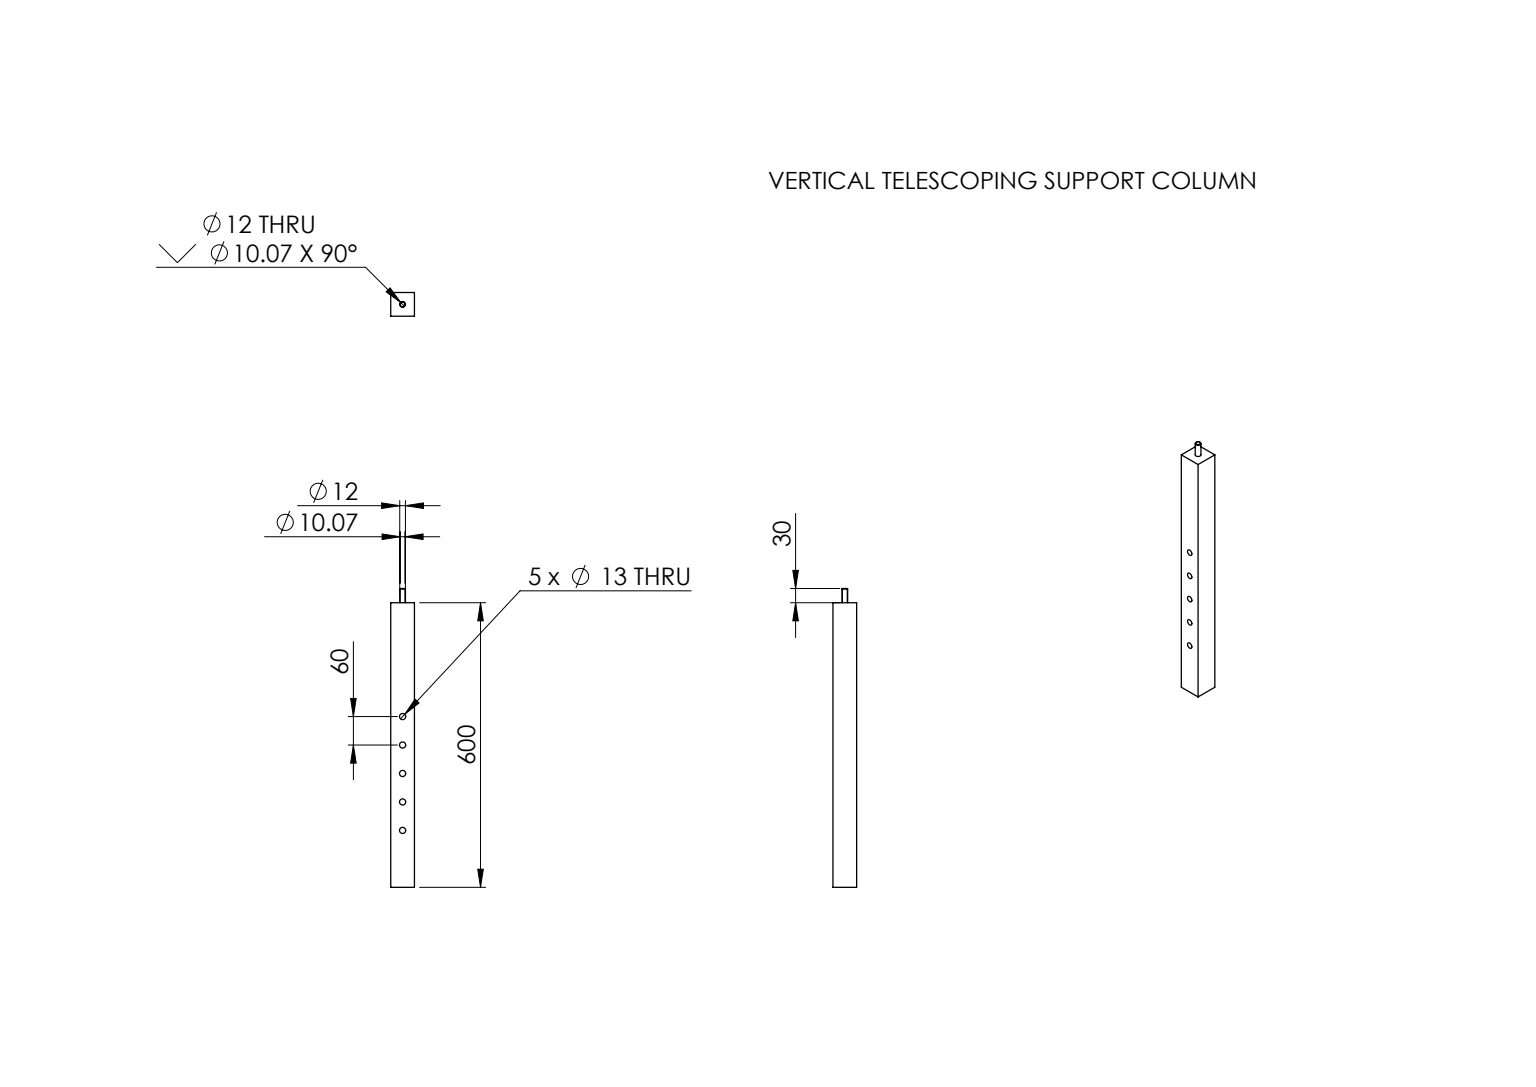
ISO-10303-21;
HEADER;
FILE_DESCRIPTION (('STEP AP214'),
    '1' );
FILE_NAME ('Vertical Telescoping Support Column.step',
    '2026-10-22T16:49:52',
    ( '' ),
    ( '' ),
    'SwSTEP 2.0',
    'SolidWorks 2026',
    '' );
FILE_SCHEMA (( 'AUTOMOTIVE_DESIGN' ));
ENDSEC;

DATA;
#19=APPLICATION_CONTEXT ( 'automotive_design' ) ;
#32=DIRECTION ( 'NONE',  ( 1.000000000000000000, -0.000000000000000000, 6.938893903907228378E-17 ) ) ;
#61=CARTESIAN_POINT ( 'NONE',  ( -24.99999999999999645, 810.0000000000000000, -25.00000000000000000 ) ) ;
#66=EDGE_LOOP ( 'NONE', ( #727, #5386, #2171, #4175 ) ) ;
#70=VECTOR ( 'NONE', #4320, 1000.000000000000000 ) ;
#84=DIRECTION ( 'NONE',  ( 2.081668171172168513E-16, 0.000000000000000000, -1.000000000000000000 ) ) ;
#89=DIRECTION ( 'NONE',  ( 1.000000000000000000, 0.000000000000000000, 0.000000000000000000 ) ) ;
#95=UNCERTAINTY_MEASURE_WITH_UNIT (LENGTH_MEASURE( 1.000000000000000082E-05 ), #3819, 'distance_accuracy_value', 'NONE');
#97=CARTESIAN_POINT ( 'NONE',  ( 0.000000000000000000, 810.0000000000000000, 0.000000000000000000 ) ) ;
#119=ADVANCED_BREP_SHAPE_REPRESENTATION ( '', ( #1812, #4154 ), #5370 ) ;
#127=DIRECTION ( 'NONE',  ( -0.000000000000000000, -0.000000000000000000, 1.000000000000000000 ) ) ;
#128=VECTOR ( 'NONE', #1979, 1000.000000000000000 ) ;
#129=CIRCLE ( 'NONE', #3889, 6.000000000000000000 ) ;
#151=ORIENTED_EDGE ( 'NONE', *, *, #3972, .F. ) ;
#161=ORIENTED_EDGE ( 'NONE', *, *, #5198, .T. ) ;
#164=DIRECTION ( 'NONE',  ( -0.000000000000000000, -0.000000000000000000, 1.000000000000000000 ) ) ;
#181=CARTESIAN_POINT ( 'NONE',  ( 0.000000000000000000, 450.0000000000000000, 25.00000000000000000 ) ) ;
#186=LINE ( 'NONE', #5103, #588 ) ;
#194=EDGE_CURVE ( 'NONE', #2394, #3572, #803, .T. ) ;
#200=ORIENTED_EDGE ( 'NONE', *, *, #4627, .T. ) ;
#204=CARTESIAN_POINT ( 'NONE',  ( 0.000000000000000000, 450.0000000000000000, -25.00000000000000000 ) ) ;
#210=CARTESIAN_POINT ( 'NONE',  ( 5.035999999999999588, 840.0000000000001137, 0.000000000000000000 ) ) ;
#217=CIRCLE ( 'NONE', #2845, 6.499999999999988454 ) ;
#223=ADVANCED_FACE ( 'NONE', ( #720 ), #3527, .F. ) ;
#226=CIRCLE ( 'NONE', #1785, 6.499999999999988454 ) ;
#237=ADVANCED_FACE ( 'NONE', ( #3202, #2295 ), #602, .T. ) ;
#253=DIRECTION ( 'NONE',  ( 1.000000000000000000, 0.000000000000000000, 0.000000000000000000 ) ) ;
#269=DIRECTION ( 'NONE',  ( 0.000000000000000000, 0.000000000000000000, -1.000000000000000000 ) ) ;
#271=CARTESIAN_POINT ( 'NONE',  ( 6.499999999999988454, 450.0000000000000000, -25.00000000000000000 ) ) ;
#325=VECTOR ( 'NONE', #1251, 1000.000000000000000 ) ;
#355=CARTESIAN_POINT ( 'NONE',  ( 0.000000000000000000, 810.0000000000000000, 0.000000000000000000 ) ) ;
#356=DIRECTION ( 'NONE',  ( 0.000000000000000000, -0.000000000000000000, 1.000000000000000000 ) ) ;
#357=DIRECTION ( 'NONE',  ( 1.000000000000000000, 0.000000000000000000, 0.000000000000000000 ) ) ;
#364=DIRECTION ( 'NONE',  ( 0.000000000000000000, 0.000000000000000000, -1.000000000000000000 ) ) ;
#393=CARTESIAN_POINT ( 'NONE',  ( -6.499999999999988454, 330.0000000000000000, 25.00000000000000000 ) ) ;
#396=ORIENTED_EDGE ( 'NONE', *, *, #1896, .F. ) ;
#398=EDGE_LOOP ( 'NONE', ( #3947, #1847, #2985, #1194 ) ) ;
#408=ADVANCED_FACE ( 'NONE', ( #4526 ), #855, .T. ) ;
#423=AXIS2_PLACEMENT_3D ( 'NONE', #2818, #3697, #3285 ) ;
#431=( LENGTH_UNIT ( ) NAMED_UNIT ( * ) SI_UNIT ( .MILLI., .METRE. ) );
#433=EDGE_CURVE ( 'NONE', #752, #1641, #4908, .T. ) ;
#448=ORIENTED_EDGE ( 'NONE', *, *, #1572, .F. ) ;
#452=ADVANCED_FACE ( 'NONE', ( #3291 ), #4007, .T. ) ;
#456=( NAMED_UNIT ( * ) SI_UNIT ( $, .STERADIAN. ) SOLID_ANGLE_UNIT ( ) );
#472=VECTOR ( 'NONE', #3512, 1000.000000000000000 ) ;
#473=EDGE_CURVE ( 'NONE', #2752, #4279, #2547, .T. ) ;
#484=AXIS2_PLACEMENT_3D ( 'NONE', #2475, #4889, #2828 ) ;
#493=PRODUCT_DEFINITION_SHAPE ( 'NONE', 'NONE',  #3566 ) ;
#497=DIRECTION ( 'NONE',  ( 0.000000000000000000, 0.000000000000000000, -1.000000000000000000 ) ) ;
#515=CARTESIAN_POINT ( 'NONE',  ( 0.000000000000000000, 840.0000000000001137, 0.000000000000000000 ) ) ;
#521=EDGE_CURVE ( 'NONE', #1452, #4077, #3495, .T. ) ;
#543=ADVANCED_FACE ( 'NONE', ( #3473 ), #4262, .F. ) ;
#550=LINE ( 'NONE', #4527, #3102 ) ;
#558=ORIENTED_EDGE ( 'NONE', *, *, #3838, .F. ) ;
#571=LINE ( 'NONE', #2235, #3982 ) ;
#573=CARTESIAN_POINT ( 'NONE',  ( 0.000000000000000000, 840.0000000000001137, 0.000000000000000000 ) ) ;
#579=ORIENTED_EDGE ( 'NONE', *, *, #4487, .F. ) ;
#582=CARTESIAN_POINT ( 'NONE',  ( -6.499999999999988454, 330.0000000000000000, 25.00000000000000000 ) ) ;
#588=VECTOR ( 'NONE', #5212, 1000.000000000000000 ) ;
#602=PLANE ( 'NONE',  #2186 ) ;
#610=EDGE_LOOP ( 'NONE', ( #4702, #3435, #2634, #3659 ) ) ;
#612=EDGE_CURVE ( 'NONE', #3569, #2957, #2707, .T. ) ;
#621=DIRECTION ( 'NONE',  ( 1.000000000000000000, 0.000000000000000000, -0.000000000000000000 ) ) ;
#629=DIRECTION ( 'NONE',  ( -0.000000000000000000, -0.000000000000000000, 1.000000000000000000 ) ) ;
#640=DIRECTION ( 'NONE',  ( -0.000000000000000000, -0.000000000000000000, 1.000000000000000000 ) ) ;
#670=AXIS2_PLACEMENT_3D ( 'NONE', #4308, #1005, #621 ) ;
#675=DIRECTION ( 'NONE',  ( 0.000000000000000000, -0.7071067811865765496, -0.7071067811865185959 ) ) ;
#682=EDGE_LOOP ( 'NONE', ( #4010, #1247, #200, #1167 ) ) ;
#693=ORIENTED_EDGE ( 'NONE', *, *, #1044, .T. ) ;
#696=DIRECTION ( 'NONE',  ( 1.000000000000000000, 0.000000000000000000, 2.081668171172168513E-16 ) ) ;
#720=FACE_OUTER_BOUND ( 'NONE', #3716, .T. ) ;
#721=DIRECTION ( 'NONE',  ( 1.000000000000000000, 0.000000000000000000, 0.000000000000000000 ) ) ;
#725=PLANE ( 'NONE',  #1977 ) ;
#727=ORIENTED_EDGE ( 'NONE', *, *, #2776, .T. ) ;
#730=CARTESIAN_POINT ( 'NONE',  ( -25.00000000000000000, 810.0000000000000000, 24.99999999999999645 ) ) ;
#744=AXIS2_PLACEMENT_3D ( 'NONE', #3308, #4537, #1587 ) ;
#746=DIRECTION ( 'NONE',  ( -0.000000000000000000, -1.000000000000000000, -0.000000000000000000 ) ) ;
#749=DIRECTION ( 'NONE',  ( 1.000000000000000000, 0.000000000000000000, 0.000000000000000000 ) ) ;
#750=CIRCLE ( 'NONE', #1517, 6.499999999999988454 ) ;
#752=VERTEX_POINT ( 'NONE', #4017 ) ;
#758=DIRECTION ( 'NONE',  ( 0.000000000000000000, 1.000000000000000000, -0.000000000000000000 ) ) ;
#759=ORIENTED_EDGE ( 'NONE', *, *, #2279, .T. ) ;
#765=ORIENTED_EDGE ( 'NONE', *, *, #433, .F. ) ;
#769=DIRECTION ( 'NONE',  ( 1.000000000000000000, 0.000000000000000000, 0.000000000000000000 ) ) ;
#770=ORIENTED_EDGE ( 'NONE', *, *, #2624, .F. ) ;
#772=EDGE_LOOP ( 'NONE', ( #4541, #1846 ) ) ;
#774=CYLINDRICAL_SURFACE ( 'NONE', #4248, 5.999999999999998224 ) ;
#780=AXIS2_PLACEMENT_3D ( 'NONE', #945, #4750, #2176 ) ;
#781=DIRECTION ( 'NONE',  ( 0.000000000000000000, -0.000000000000000000, 1.000000000000000000 ) ) ;
#782=ORIENTED_EDGE ( 'NONE', *, *, #5242, .T. ) ;
#791=VERTEX_POINT ( 'NONE', #4572 ) ;
#803=CIRCLE ( 'NONE', #1475, 6.499999999999988454 ) ;
#806=CARTESIAN_POINT ( 'NONE',  ( 0.000000000000000000, 839.0360000000000582, 0.000000000000000000 ) ) ;
#816=ORIENTED_EDGE ( 'NONE', *, *, #5242, .F. ) ;
#838=VERTEX_POINT ( 'NONE', #4461 ) ;
#855=CYLINDRICAL_SURFACE ( 'NONE', #1148, 5.999999999999998224 ) ;
#869=EDGE_LOOP ( 'NONE', ( #1482, #1899, #1551, #4613 ) ) ;
#871=VERTEX_POINT ( 'NONE', #2071 ) ;
#872=FACE_OUTER_BOUND ( 'NONE', #66, .T. ) ;
#877=FACE_OUTER_BOUND ( 'NONE', #4794, .T. ) ;
#881=CARTESIAN_POINT ( 'NONE',  ( 25.00000000000000000, 210.0000000000000284, -25.00000000000000000 ) ) ;
#901=VECTOR ( 'NONE', #2965, 1000.000000000000000 ) ;
#910=STYLED_ITEM ( 'NONE', ( #4984 ), #119 ) ;
#914=FACE_BOUND ( 'NONE', #4721, .T. ) ;
#930=ADVANCED_FACE ( 'NONE', ( #914, #5090, #872, #3823, #2115, #1280 ), #5121, .F. ) ;
#931=CIRCLE ( 'NONE', #3993, 6.499999999999988454 ) ;
#934=DIRECTION ( 'NONE',  ( -1.000000000000000000, 0.000000000000000000, 0.000000000000000000 ) ) ;
#942=( NAMED_UNIT ( * ) SI_UNIT ( $, .STERADIAN. ) SOLID_ANGLE_UNIT ( ) );
#944=DIRECTION ( 'NONE',  ( -1.000000000000000000, 0.000000000000000000, -2.081668171172168513E-16 ) ) ;
#945=CARTESIAN_POINT ( 'NONE',  ( 0.000000000000000000, 510.0000000000000000, 25.00000000000000000 ) ) ;
#956=CARTESIAN_POINT ( 'NONE',  ( -24.99999999999999645, 210.0000000000000284, -25.00000000000000000 ) ) ;
#971=CARTESIAN_POINT ( 'NONE',  ( 0.000000000000000000, 570.0000000000000000, -25.00000000000000000 ) ) ;
#975=DIRECTION ( 'NONE',  ( 1.000000000000000000, 0.000000000000000000, 0.000000000000000000 ) ) ;
#985=CARTESIAN_POINT ( 'NONE',  ( 0.000000000000000000, 810.0000000000000000, 0.000000000000000000 ) ) ;
#986=DIRECTION ( 'NONE',  ( -0.000000000000000000, -0.000000000000000000, 1.000000000000000000 ) ) ;
#988=CARTESIAN_POINT ( 'NONE',  ( 0.000000000000000000, 570.0000000000000000, 25.00000000000000000 ) ) ;
#989=VECTOR ( 'NONE', #1784, 1000.000000000000000 ) ;
#991=ORIENTED_EDGE ( 'NONE', *, *, #4856, .T. ) ;
#1005=DIRECTION ( 'NONE',  ( 0.000000000000000000, -0.000000000000000000, 1.000000000000000000 ) ) ;
#1007=ORIENTED_EDGE ( 'NONE', *, *, #2705, .F. ) ;
#1024=LINE ( 'NONE', #1388, #1958 ) ;
#1044=EDGE_CURVE ( 'NONE', #3246, #871, #5265, .T. ) ;
#1051=CARTESIAN_POINT ( 'NONE',  ( -24.99999999999999645, 810.0000000000000000, -25.00000000000000000 ) ) ;
#1052=ORIENTED_EDGE ( 'NONE', *, *, #4879, .T. ) ;
#1059=ORIENTED_EDGE ( 'NONE', *, *, #1669, .T. ) ;
#1068=LINE ( 'NONE', #2631, #4741 ) ;
#1096=CARTESIAN_POINT ( 'NONE',  ( 0.000000000000000000, 810.0000000000000000, -6.000000000000000000 ) ) ;
#1097=DIRECTION ( 'NONE',  ( 1.000000000000000000, 0.000000000000000000, 0.000000000000000000 ) ) ;
#1099=DIRECTION ( 'NONE',  ( 0.000000000000000000, -0.000000000000000000, 1.000000000000000000 ) ) ;
#1123=ORIENTED_EDGE ( 'NONE', *, *, #5224, .F. ) ;
#1129=DIRECTION ( 'NONE',  ( -6.938893903907228378E-17, 0.000000000000000000, 1.000000000000000000 ) ) ;
#1142=ORIENTED_EDGE ( 'NONE', *, *, #1592, .T. ) ;
#1148=AXIS2_PLACEMENT_3D ( 'NONE', #1996, #2445, #4184 ) ;
#1157=ORIENTED_EDGE ( 'NONE', *, *, #2641, .T. ) ;
#1160=VERTEX_POINT ( 'NONE', #1839 ) ;
#1165=FACE_OUTER_BOUND ( 'NONE', #2433, .T. ) ;
#1167=ORIENTED_EDGE ( 'NONE', *, *, #521, .T. ) ;
#1181=DIRECTION ( 'NONE',  ( 1.000000000000000000, 0.000000000000000000, 0.000000000000000000 ) ) ;
#1185=MECHANICAL_DESIGN_GEOMETRIC_PRESENTATION_REPRESENTATION('',(#910),#2945);
#1189=EDGE_LOOP ( 'NONE', ( #3290, #4950 ) ) ;
#1194=ORIENTED_EDGE ( 'NONE', *, *, #2265, .T. ) ;
#1200=EDGE_LOOP ( 'NONE', ( #2737, #2902, #4173, #4013 ) ) ;
#1201=CIRCLE ( 'NONE', #2515, 6.499999999999988454 ) ;
#1211=VECTOR ( 'NONE', #2256, 1000.000000000000000 ) ;
#1212=EDGE_CURVE ( 'NONE', #4428, #4561, #3545, .T. ) ;
#1216=CARTESIAN_POINT ( 'NONE',  ( 25.00000000000000000, 210.0000000000000284, 25.00000000000000711 ) ) ;
#1218=EDGE_CURVE ( 'NONE', #4553, #3240, #5228, .T. ) ;
#1246=CARTESIAN_POINT ( 'NONE',  ( 0.000000000000000000, 330.0000000000000000, 25.00000000000000000 ) ) ;
#1247=ORIENTED_EDGE ( 'NONE', *, *, #2005, .T. ) ;
#1251=DIRECTION ( 'NONE',  ( -0.000000000000000000, -1.000000000000000000, -0.000000000000000000 ) ) ;
#1262=ORIENTED_EDGE ( 'NONE', *, *, #2641, .F. ) ;
#1274=EDGE_LOOP ( 'NONE', ( #1059, #1123, #2107, #2096 ) ) ;
#1276=AXIS2_PLACEMENT_3D ( 'NONE', #4113, #3259, #721 ) ;
#1279=VERTEX_POINT ( 'NONE', #2369 ) ;
#1280=FACE_BOUND ( 'NONE', #2660, .T. ) ;
#1291=AXIS2_PLACEMENT_3D ( 'NONE', #1570, #4441, #3252 ) ;
#1302=ORIENTED_EDGE ( 'NONE', *, *, #3286, .F. ) ;
#1330=ORIENTED_EDGE ( 'NONE', *, *, #4981, .F. ) ;
#1331=ADVANCED_FACE ( 'NONE', ( #877 ), #1376, .F. ) ;
#1340=CIRCLE ( 'NONE', #2041, 6.499999999999988454 ) ;
#1355=CIRCLE ( 'NONE', #2063, 6.499999999999988454 ) ;
#1360=CARTESIAN_POINT ( 'NONE',  ( 0.000000000000000000, 330.0000000000000000, -25.00000000000000000 ) ) ;
#1368=CARTESIAN_POINT ( 'NONE',  ( 7.347880794884119736E-16, 810.0000000000000000, 6.000000000000000000 ) ) ;
#1369=CIRCLE ( 'NONE', #4508, 6.499999999999988454 ) ;
#1376=PLANE ( 'NONE',  #1851 ) ;
#1378=DIRECTION ( 'NONE',  ( -0.000000000000000000, -1.000000000000000000, -0.000000000000000000 ) ) ;
#1383=CARTESIAN_POINT ( 'NONE',  ( 0.000000000000000000, 570.0000000000000000, 25.00000000000000000 ) ) ;
#1385=LINE ( 'NONE', #582, #1966 ) ;
#1386=CARTESIAN_POINT ( 'NONE',  ( -6.499999999999988454, 510.0000000000000000, 25.00000000000000000 ) ) ;
#1388=CARTESIAN_POINT ( 'NONE',  ( -6.499999999999988454, 570.0000000000000000, 25.00000000000000000 ) ) ;
#1394=CARTESIAN_POINT ( 'NONE',  ( -24.99999999999999645, 810.0000000000000000, -25.00000000000000000 ) ) ;
#1400=CARTESIAN_POINT ( 'NONE',  ( 6.499999999999988454, 330.0000000000000000, 25.00000000000000000 ) ) ;
#1409=DIRECTION ( 'NONE',  ( -0.000000000000000000, -0.000000000000000000, 1.000000000000000000 ) ) ;
#1415=CIRCLE ( 'NONE', #3532, 5.999999999999996447 ) ;
#1446=AXIS2_PLACEMENT_3D ( 'NONE', #573, #5179, #4342 ) ;
#1448=AXIS2_PLACEMENT_3D ( 'NONE', #181, #127, #3847 ) ;
#1452=VERTEX_POINT ( 'NONE', #2735 ) ;
#1475=AXIS2_PLACEMENT_3D ( 'NONE', #1383, #4705, #2656 ) ;
#1482=ORIENTED_EDGE ( 'NONE', *, *, #2888, .F. ) ;
#1485=CARTESIAN_POINT ( 'NONE',  ( 0.000000000000000000, 450.0000000000000000, 25.00000000000000000 ) ) ;
#1497=CARTESIAN_POINT ( 'NONE',  ( 0.000000000000000000, 330.0000000000000000, 25.00000000000000000 ) ) ;
#1516=CARTESIAN_POINT ( 'NONE',  ( 0.000000000000000000, 839.0360000000000582, -5.999999999999996447 ) ) ;
#1517=AXIS2_PLACEMENT_3D ( 'NONE', #2658, #1099, #3485 ) ;
#1535=ORIENTED_EDGE ( 'NONE', *, *, #1218, .F. ) ;
#1536=CIRCLE ( 'NONE', #2599, 6.499999999999988454 ) ;
#1542=CIRCLE ( 'NONE', #2523, 6.499999999999988454 ) ;
#1546=FACE_OUTER_BOUND ( 'NONE', #3238, .T. ) ;
#1548=UNCERTAINTY_MEASURE_WITH_UNIT (LENGTH_MEASURE( 1.000000000000000082E-05 ), #1640, 'distance_accuracy_value', 'NONE');
#1551=ORIENTED_EDGE ( 'NONE', *, *, #612, .F. ) ;
#1561=VERTEX_POINT ( 'NONE', #1096 ) ;
#1563=DIRECTION ( 'NONE',  ( -0.000000000000000000, -1.000000000000000000, -0.000000000000000000 ) ) ;
#1570=CARTESIAN_POINT ( 'NONE',  ( 0.000000000000000000, 839.0360000000000582, 0.000000000000000000 ) ) ;
#1572=EDGE_CURVE ( 'NONE', #4239, #4335, #2381, .T. ) ;
#1574=LINE ( 'NONE', #4905, #3175 ) ;
#1575=VERTEX_POINT ( 'NONE', #2768 ) ;
#1581=EDGE_LOOP ( 'NONE', ( #3949, #2582, #4492, #2380 ) ) ;
#1587=DIRECTION ( 'NONE',  ( 1.000000000000000000, 0.000000000000000000, 0.000000000000000000 ) ) ;
#1592=EDGE_CURVE ( 'NONE', #752, #3517, #1340, .T. ) ;
#1610=VECTOR ( 'NONE', #5101, 1000.000000000000000 ) ;
#1616=ORIENTED_EDGE ( 'NONE', *, *, #5060, .T. ) ;
#1625=ORIENTED_EDGE ( 'NONE', *, *, #5027, .F. ) ;
#1629=VECTOR ( 'NONE', #364, 1000.000000000000000 ) ;
#1639=CIRCLE ( 'NONE', #2609, 6.499999999999988454 ) ;
#1640=( LENGTH_UNIT ( ) NAMED_UNIT ( * ) SI_UNIT ( .MILLI., .METRE. ) );
#1641=VERTEX_POINT ( 'NONE', #4054 ) ;
#1648=EDGE_LOOP ( 'NONE', ( #1052, #3103 ) ) ;
#1649=EDGE_LOOP ( 'NONE', ( #2000, #1142 ) ) ;
#1652=ORIENTED_EDGE ( 'NONE', *, *, #194, .F. ) ;
#1654=LINE ( 'NONE', #730, #128 ) ;
#1669=EDGE_CURVE ( 'NONE', #2957, #3489, #1574, .T. ) ;
#1671=ORIENTED_EDGE ( 'NONE', *, *, #1572, .T. ) ;
#1703=EDGE_LOOP ( 'NONE', ( #4334, #4590 ) ) ;
#1719=DIRECTION ( 'NONE',  ( 6.938893903907228378E-17, 0.000000000000000000, -1.000000000000000000 ) ) ;
#1736=EDGE_CURVE ( 'NONE', #2365, #1561, #3051, .T. ) ;
#1749=PRODUCT ( 'Vertical Telescoping Support Column', 'Vertical Telescoping Support Column', '', ( #4877 ) ) ;
#1751=ORIENTED_EDGE ( 'NONE', *, *, #5316, .F. ) ;
#1766=FACE_BOUND ( 'NONE', #4681, .T. ) ;
#1776=FACE_OUTER_BOUND ( 'NONE', #2546, .T. ) ;
#1781=AXIS2_PLACEMENT_3D ( 'NONE', #3811, #934, #3785 ) ;
#1784=DIRECTION ( 'NONE',  ( -0.000000000000000000, -1.000000000000000000, -0.000000000000000000 ) ) ;
#1785=AXIS2_PLACEMENT_3D ( 'NONE', #2894, #3616, #1181 ) ;
#1788=DIRECTION ( 'NONE',  ( 1.000000000000000000, 0.000000000000000000, 0.000000000000000000 ) ) ;
#1799=FACE_OUTER_BOUND ( 'NONE', #1581, .T. ) ;
#1807=DIRECTION ( 'NONE',  ( -0.000000000000000000, -1.000000000000000000, -0.000000000000000000 ) ) ;
#1812=MANIFOLD_SOLID_BREP ( 'LPattern1', #5093 ) ;
#1821=DIRECTION ( 'NONE',  ( 1.000000000000000000, 0.000000000000000000, 0.000000000000000000 ) ) ;
#1824=ORIENTED_EDGE ( 'NONE', *, *, #4857, .F. ) ;
#1830=FACE_OUTER_BOUND ( 'NONE', #3347, .T. ) ;
#1839=CARTESIAN_POINT ( 'NONE',  ( -25.00000000000000000, 810.0000000000000000, 24.99999999999999645 ) ) ;
#1846=ORIENTED_EDGE ( 'NONE', *, *, #2792, .F. ) ;
#1847=ORIENTED_EDGE ( 'NONE', *, *, #473, .F. ) ;
#1849=CARTESIAN_POINT ( 'NONE',  ( 0.000000000000000000, 330.0000000000000000, 25.00000000000000000 ) ) ;
#1850=CARTESIAN_POINT ( 'NONE',  ( -6.499999999999988454, 450.0000000000000000, -25.00000000000000000 ) ) ;
#1851=AXIS2_PLACEMENT_3D ( 'NONE', #61, #32, #1719 ) ;
#1855=( GEOMETRIC_REPRESENTATION_CONTEXT ( 3 ) GLOBAL_UNCERTAINTY_ASSIGNED_CONTEXT ( ( #1548 ) ) GLOBAL_UNIT_ASSIGNED_CONTEXT ( ( #1640, #4964, #942 ) ) REPRESENTATION_CONTEXT ( 'NONE', 'WORKASPACE' ) );
#1858=AXIS2_PLACEMENT_3D ( 'NONE', #97, #5041, #3433 ) ;
#1870=FACE_BOUND ( 'NONE', #1649, .T. ) ;
#1885=CONICAL_SURFACE ( 'NONE', #3031, 5.999999999999996447, 0.7853981633974074228 ) ;
#1896=EDGE_CURVE ( 'NONE', #3246, #2365, #2308, .T. ) ;
#1899=ORIENTED_EDGE ( 'NONE', *, *, #1669, .F. ) ;
#1906=CARTESIAN_POINT ( 'NONE',  ( 0.000000000000000000, 390.0000000000000000, -25.00000000000000000 ) ) ;
#1926=ADVANCED_FACE ( 'NONE', ( #5318 ), #2399, .F. ) ;
#1932=CARTESIAN_POINT ( 'NONE',  ( 6.499999999999988454, 570.0000000000000000, 25.00000000000000000 ) ) ;
#1933=CARTESIAN_POINT ( 'NONE',  ( 6.499999999999988454, 390.0000000000000000, 25.00000000000000000 ) ) ;
#1958=VECTOR ( 'NONE', #4709, 1000.000000000000000 ) ;
#1964=LINE ( 'NONE', #3205, #4075 ) ;
#1966=VECTOR ( 'NONE', #3068, 1000.000000000000000 ) ;
#1977=AXIS2_PLACEMENT_3D ( 'NONE', #2390, #758, #2865 ) ;
#1979=DIRECTION ( 'NONE',  ( 1.000000000000000000, 0.000000000000000000, 2.081668171172168513E-16 ) ) ;
#1980=EDGE_CURVE ( 'NONE', #2365, #4239, #1415, .T. ) ;
#1988=CARTESIAN_POINT ( 'NONE',  ( 0.000000000000000000, 330.0000000000000000, 25.00000000000000000 ) ) ;
#1996=CARTESIAN_POINT ( 'NONE',  ( 0.000000000000000000, 810.0000000000000000, 0.000000000000000000 ) ) ;
#1999=ORIENTED_EDGE ( 'NONE', *, *, #2888, .T. ) ;
#2000=ORIENTED_EDGE ( 'NONE', *, *, #4597, .T. ) ;
#2005=EDGE_CURVE ( 'NONE', #1160, #2006, #1654, .T. ) ;
#2006=VERTEX_POINT ( 'NONE', #3768 ) ;
#2020=CARTESIAN_POINT ( 'NONE',  ( -6.499999999999988454, 390.0000000000000000, 25.00000000000000000 ) ) ;
#2041=AXIS2_PLACEMENT_3D ( 'NONE', #1906, #781, #4085 ) ;
#2051=ADVANCED_FACE ( 'NONE', ( #1165 ), #2929, .F. ) ;
#2052=CARTESIAN_POINT ( 'NONE',  ( 0.000000000000000000, 390.0000000000000000, -25.00000000000000000 ) ) ;
#2063=AXIS2_PLACEMENT_3D ( 'NONE', #3735, #5075, #89 ) ;
#2064=DIRECTION ( 'NONE',  ( 0.000000000000000000, 0.000000000000000000, -1.000000000000000000 ) ) ;
#2071=CARTESIAN_POINT ( 'NONE',  ( 6.757601037695092606E-16, 840.0000000000001137, 5.035999999999999588 ) ) ;
#2096=ORIENTED_EDGE ( 'NONE', *, *, #3480, .T. ) ;
#2107=ORIENTED_EDGE ( 'NONE', *, *, #521, .F. ) ;
#2115=FACE_BOUND ( 'NONE', #772, .T. ) ;
#2116=CARTESIAN_POINT ( 'NONE',  ( 25.00000000000000000, 810.0000000000000000, 25.00000000000000711 ) ) ;
#2141=SURFACE_STYLE_FILL_AREA ( #2457 ) ;
#2154=DIRECTION ( 'NONE',  ( 1.000000000000000000, 0.000000000000000000, 0.000000000000000000 ) ) ;
#2160=EDGE_CURVE ( 'NONE', #1561, #4335, #4227, .T. ) ;
#2161=CIRCLE ( 'NONE', #2880, 6.499999999999988454 ) ;
#2171=ORIENTED_EDGE ( 'NONE', *, *, #2005, .F. ) ;
#2176=DIRECTION ( 'NONE',  ( 1.000000000000000000, 0.000000000000000000, 0.000000000000000000 ) ) ;
#2186=AXIS2_PLACEMENT_3D ( 'NONE', #3964, #4419, #3938 ) ;
#2193=DIRECTION ( 'NONE',  ( -0.000000000000000000, -0.000000000000000000, 1.000000000000000000 ) ) ;
#2215=DIRECTION ( 'NONE',  ( -0.000000000000000000, -1.000000000000000000, -0.000000000000000000 ) ) ;
#2217=CARTESIAN_POINT ( 'NONE',  ( 0.000000000000000000, 839.0360000000000582, 0.000000000000000000 ) ) ;
#2235=CARTESIAN_POINT ( 'NONE',  ( 6.499999999999988454, 450.0000000000000000, 25.00000000000000000 ) ) ;
#2246=CARTESIAN_POINT ( 'NONE',  ( 6.499999999999988454, 330.0000000000000000, -25.00000000000000000 ) ) ;
#2251=( NAMED_UNIT ( * ) PLANE_ANGLE_UNIT ( ) SI_UNIT ( $, .RADIAN. ) );
#2256=DIRECTION ( 'NONE',  ( -0.000000000000000000, -1.000000000000000000, -0.000000000000000000 ) ) ;
#2261=FACE_BOUND ( 'NONE', #4304, .T. ) ;
#2263=DIRECTION ( 'NONE',  ( 1.000000000000000000, 0.000000000000000000, 0.000000000000000000 ) ) ;
#2265=EDGE_CURVE ( 'NONE', #3572, #2394, #217, .T. ) ;
#2270=CYLINDRICAL_SURFACE ( 'NONE', #3188, 6.499999999999988454 ) ;
#2279=EDGE_CURVE ( 'NONE', #4279, #2394, #1024, .T. ) ;
#2295=FACE_OUTER_BOUND ( 'NONE', #682, .T. ) ;
#2297=DIRECTION ( 'NONE',  ( 0.000000000000000000, 0.000000000000000000, -1.000000000000000000 ) ) ;
#2304=ORIENTED_EDGE ( 'NONE', *, *, #3972, .T. ) ;
#2308=LINE ( 'NONE', #4014, #2663 ) ;
#2321=CIRCLE ( 'NONE', #3024, 6.499999999999988454 ) ;
#2339=AXIS2_PLACEMENT_3D ( 'NONE', #806, #1378, #497 ) ;
#2365=VERTEX_POINT ( 'NONE', #1516 ) ;
#2369=CARTESIAN_POINT ( 'NONE',  ( 6.499999999999988454, 510.0000000000000000, 25.00000000000000000 ) ) ;
#2376=DIRECTION ( 'NONE',  ( -0.000000000000000000, -0.000000000000000000, 1.000000000000000000 ) ) ;
#2380=ORIENTED_EDGE ( 'NONE', *, *, #4566, .F. ) ;
#2381=LINE ( 'NONE', #2443, #4305 ) ;
#2383=CARTESIAN_POINT ( 'NONE',  ( 0.000000000000000000, 450.0000000000000000, 25.00000000000000000 ) ) ;
#2390=CARTESIAN_POINT ( 'NONE',  ( 0.000000000000000000, 210.0000000000000284, 0.000000000000000000 ) ) ;
#2391=ADVANCED_FACE ( 'NONE', ( #3620 ), #2899, .F. ) ;
#2394=VERTEX_POINT ( 'NONE', #2505 ) ;
#2399=CYLINDRICAL_SURFACE ( 'NONE', #744, 6.499999999999988454 ) ;
#2424=ORIENTED_EDGE ( 'NONE', *, *, #473, .T. ) ;
#2433=EDGE_LOOP ( 'NONE', ( #1007, #3544, #2793, #1157 ) ) ;
#2434=CARTESIAN_POINT ( 'NONE',  ( 0.000000000000000000, 0.000000000000000000, 0.000000000000000000 ) ) ;
#2438=VERTEX_POINT ( 'NONE', #393 ) ;
#2440=DIRECTION ( 'NONE',  ( -0.000000000000000000, -1.000000000000000000, -0.000000000000000000 ) ) ;
#2443=CARTESIAN_POINT ( 'NONE',  ( 7.347880794884117764E-16, 810.0000000000000000, 5.999999999999998224 ) ) ;
#2445=DIRECTION ( 'NONE',  ( -0.000000000000000000, -1.000000000000000000, -0.000000000000000000 ) ) ;
#2457=FILL_AREA_STYLE ('',( #3334 ) ) ;
#2475=CARTESIAN_POINT ( 'NONE',  ( 0.000000000000000000, 450.0000000000000000, 25.00000000000000000 ) ) ;
#2479=ORIENTED_EDGE ( 'NONE', *, *, #2160, .F. ) ;
#2493=ADVANCED_FACE ( 'NONE', ( #3761 ), #4611, .F. ) ;
#2501=COLOUR_RGB ( '',0.8941176470588234615, 0.8941176470588234615, 0.8941176470588234615 ) ;
#2505=CARTESIAN_POINT ( 'NONE',  ( -6.499999999999988454, 570.0000000000000000, 25.00000000000000000 ) ) ;
#2506=UNCERTAINTY_MEASURE_WITH_UNIT (LENGTH_MEASURE( 1.000000000000000082E-05 ), #431, 'distance_accuracy_value', 'NONE');
#2515=AXIS2_PLACEMENT_3D ( 'NONE', #1485, #4106, #5296 ) ;
#2521=LINE ( 'NONE', #2116, #325 ) ;
#2523=AXIS2_PLACEMENT_3D ( 'NONE', #1360, #4386, #2263 ) ;
#2535=ORIENTED_EDGE ( 'NONE', *, *, #2705, .T. ) ;
#2546=EDGE_LOOP ( 'NONE', ( #3922, #3951, #2593, #151 ) ) ;
#2547=CIRCLE ( 'NONE', #3000, 6.499999999999988454 ) ;
#2574=CARTESIAN_POINT ( 'NONE',  ( 0.000000000000000000, 570.0000000000000000, 25.00000000000000000 ) ) ;
#2581=ADVANCED_FACE ( 'NONE', ( #1830 ), #2270, .F. ) ;
#2582=ORIENTED_EDGE ( 'NONE', *, *, #433, .T. ) ;
#2593=ORIENTED_EDGE ( 'NONE', *, *, #4981, .T. ) ;
#2596=DIRECTION ( 'NONE',  ( 1.000000000000000000, 0.000000000000000000, 0.000000000000000000 ) ) ;
#2599=AXIS2_PLACEMENT_3D ( 'NONE', #1497, #4686, #3069 ) ;
#2604=FACE_OUTER_BOUND ( 'NONE', #1189, .T. ) ;
#2609=AXIS2_PLACEMENT_3D ( 'NONE', #4275, #3492, #2596 ) ;
#2621=EDGE_CURVE ( 'NONE', #4335, #1561, #129, .T. ) ;
#2624=EDGE_CURVE ( 'NONE', #2728, #4553, #750, .T. ) ;
#2631=CARTESIAN_POINT ( 'NONE',  ( 25.00000000000000000, 810.0000000000000000, -25.00000000000000000 ) ) ;
#2634=ORIENTED_EDGE ( 'NONE', *, *, #1896, .T. ) ;
#2641=EDGE_CURVE ( 'NONE', #3240, #2438, #2944, .T. ) ;
#2647=CARTESIAN_POINT ( 'NONE',  ( 25.00000000000000000, 810.0000000000000000, -25.00000000000000000 ) ) ;
#2648=FACE_OUTER_BOUND ( 'NONE', #1274, .T. ) ;
#2656=DIRECTION ( 'NONE',  ( 1.000000000000000000, 0.000000000000000000, 0.000000000000000000 ) ) ;
#2658=CARTESIAN_POINT ( 'NONE',  ( 0.000000000000000000, 330.0000000000000000, -25.00000000000000000 ) ) ;
#2659=LINE ( 'NONE', #1386, #70 ) ;
#2660=EDGE_LOOP ( 'NONE', ( #1262, #2891 ) ) ;
#2663=VECTOR ( 'NONE', #675, 999.9999999999998863 ) ;
#2667=ORIENTED_EDGE ( 'NONE', *, *, #1736, .T. ) ;
#2676=EDGE_LOOP ( 'NONE', ( #448, #1616, #2667, #5000 ) ) ;
#2697=DIRECTION ( 'NONE',  ( -0.000000000000000000, -0.000000000000000000, 1.000000000000000000 ) ) ;
#2703=CARTESIAN_POINT ( 'NONE',  ( -6.499999999999988454, 450.0000000000000000, 25.00000000000000000 ) ) ;
#2705=EDGE_CURVE ( 'NONE', #2728, #2438, #1385, .T. ) ;
#2707=LINE ( 'NONE', #5208, #3707 ) ;
#2728=VERTEX_POINT ( 'NONE', #4767 ) ;
#2729=EDGE_LOOP ( 'NONE', ( #3248, #1671, #2479, #4809 ) ) ;
#2733=DIRECTION ( 'NONE',  ( 1.000000000000000000, 0.000000000000000000, 0.000000000000000000 ) ) ;
#2735=CARTESIAN_POINT ( 'NONE',  ( 25.00000000000000000, 810.0000000000000000, -25.00000000000000000 ) ) ;
#2737=ORIENTED_EDGE ( 'NONE', *, *, #612, .T. ) ;
#2752=VERTEX_POINT ( 'NONE', #5249 ) ;
#2762=AXIS2_PLACEMENT_3D ( 'NONE', #2574, #4232, #2154 ) ;
#2768=CARTESIAN_POINT ( 'NONE',  ( -25.00000000000000000, 210.0000000000000284, 24.99999999999999645 ) ) ;
#2776=EDGE_CURVE ( 'NONE', #1575, #3569, #550, .T. ) ;
#2792=EDGE_CURVE ( 'NONE', #1641, #2863, #3019, .T. ) ;
#2793=ORIENTED_EDGE ( 'NONE', *, *, #1218, .T. ) ;
#2818=CARTESIAN_POINT ( 'NONE',  ( 0.000000000000000000, 510.0000000000000000, -25.00000000000000000 ) ) ;
#2821=DIRECTION ( 'NONE',  ( -0.000000000000000000, -0.000000000000000000, 1.000000000000000000 ) ) ;
#2828=DIRECTION ( 'NONE',  ( 1.000000000000000000, 0.000000000000000000, 0.000000000000000000 ) ) ;
#2845=AXIS2_PLACEMENT_3D ( 'NONE', #988, #2697, #3567 ) ;
#2863=VERTEX_POINT ( 'NONE', #1933 ) ;
#2865=DIRECTION ( 'NONE',  ( 0.000000000000000000, 0.000000000000000000, 1.000000000000000000 ) ) ;
#2871=ORIENTED_EDGE ( 'NONE', *, *, #5198, .F. ) ;
#2876=EDGE_CURVE ( 'NONE', #4428, #4982, #226, .T. ) ;
#2879=( NAMED_UNIT ( * ) PLANE_ANGLE_UNIT ( ) SI_UNIT ( $, .RADIAN. ) );
#2880=AXIS2_PLACEMENT_3D ( 'NONE', #204, #5171, #1788 ) ;
#2883=LINE ( 'NONE', #4573, #5112 ) ;
#2888=EDGE_CURVE ( 'NONE', #3489, #1575, #1964, .T. ) ;
#2891=ORIENTED_EDGE ( 'NONE', *, *, #4540, .F. ) ;
#2894=CARTESIAN_POINT ( 'NONE',  ( 0.000000000000000000, 450.0000000000000000, -25.00000000000000000 ) ) ;
#2895=LINE ( 'NONE', #4528, #1629 ) ;
#2899=CYLINDRICAL_SURFACE ( 'NONE', #484, 6.499999999999988454 ) ;
#2901=ORIENTED_EDGE ( 'NONE', *, *, #3232, .F. ) ;
#2902=ORIENTED_EDGE ( 'NONE', *, *, #3480, .F. ) ;
#2929=CYLINDRICAL_SURFACE ( 'NONE', #4396, 6.499999999999988454 ) ;
#2933=ORIENTED_EDGE ( 'NONE', *, *, #3232, .T. ) ;
#2944=CIRCLE ( 'NONE', #5016, 6.499999999999988454 ) ;
#2945=( GEOMETRIC_REPRESENTATION_CONTEXT ( 3 ) GLOBAL_UNCERTAINTY_ASSIGNED_CONTEXT ( ( #2506 ) ) GLOBAL_UNIT_ASSIGNED_CONTEXT ( ( #431, #2251, #4710 ) ) REPRESENTATION_CONTEXT ( 'NONE', 'WORKASPACE' ) );
#2952=CARTESIAN_POINT ( 'NONE',  ( 0.000000000000000000, 510.0000000000000000, 25.00000000000000000 ) ) ;
#2957=VERTEX_POINT ( 'NONE', #881 ) ;
#2959=VECTOR ( 'NONE', #986, 1000.000000000000000 ) ;
#2965=DIRECTION ( 'NONE',  ( -1.000000000000000000, 0.000000000000000000, 0.000000000000000000 ) ) ;
#2969=EDGE_CURVE ( 'NONE', #1160, #1575, #4626, .T. ) ;
#2973=EDGE_LOOP ( 'NONE', ( #579, #1625, #2304, #161 ) ) ;
#2985=ORIENTED_EDGE ( 'NONE', *, *, #4857, .T. ) ;
#3000=AXIS2_PLACEMENT_3D ( 'NONE', #971, #5099, #1821 ) ;
#3019=CIRCLE ( 'NONE', #1276, 6.499999999999988454 ) ;
#3024=AXIS2_PLACEMENT_3D ( 'NONE', #4107, #356, #4933 ) ;
#3031=AXIS2_PLACEMENT_3D ( 'NONE', #2217, #5220, #4394 ) ;
#3037=DIRECTION ( 'NONE',  ( -0.000000000000000000, -0.000000000000000000, 1.000000000000000000 ) ) ;
#3042=CARTESIAN_POINT ( 'NONE',  ( 6.499999999999988454, 390.0000000000000000, -25.00000000000000000 ) ) ;
#3051=LINE ( 'NONE', #4254, #989 ) ;
#3061=CARTESIAN_POINT ( 'NONE',  ( 0.000000000000000000, 390.0000000000000000, 25.00000000000000000 ) ) ;
#3068=DIRECTION ( 'NONE',  ( -0.000000000000000000, -0.000000000000000000, 1.000000000000000000 ) ) ;
#3069=DIRECTION ( 'NONE',  ( 1.000000000000000000, 0.000000000000000000, 0.000000000000000000 ) ) ;
#3075=CARTESIAN_POINT ( 'NONE',  ( 6.499999999999988454, 330.0000000000000000, 25.00000000000000000 ) ) ;
#3080=DIRECTION ( 'NONE',  ( 0.000000000000000000, 0.000000000000000000, -1.000000000000000000 ) ) ;
#3081=DIRECTION ( 'NONE',  ( 0.000000000000000000, -0.000000000000000000, 1.000000000000000000 ) ) ;
#3102=VECTOR ( 'NONE', #696, 1000.000000000000000 ) ;
#3103=ORIENTED_EDGE ( 'NONE', *, *, #2624, .T. ) ;
#3110=ORIENTED_EDGE ( 'NONE', *, *, #1212, .T. ) ;
#3113=PLANE ( 'NONE',  #670 ) ;
#3159=FACE_OUTER_BOUND ( 'NONE', #2676, .T. ) ;
#3172=AXIS2_PLACEMENT_3D ( 'NONE', #515, #4224, #5067 ) ;
#3175=VECTOR ( 'NONE', #5304, 1000.000000000000000 ) ;
#3188=AXIS2_PLACEMENT_3D ( 'NONE', #3887, #629, #3562 ) ;
#3202=FACE_BOUND ( 'NONE', #1703, .T. ) ;
#3205=CARTESIAN_POINT ( 'NONE',  ( -24.99999999999999645, 210.0000000000000284, -25.00000000000000000 ) ) ;
#3232=EDGE_CURVE ( 'NONE', #4982, #791, #571, .T. ) ;
#3238=EDGE_LOOP ( 'NONE', ( #770, #2535, #4482, #1535 ) ) ;
#3240=VERTEX_POINT ( 'NONE', #1400 ) ;
#3246=VERTEX_POINT ( 'NONE', #5349 ) ;
#3247=ORIENTED_EDGE ( 'NONE', *, *, #4597, .F. ) ;
#3248=ORIENTED_EDGE ( 'NONE', *, *, #1980, .T. ) ;
#3252=DIRECTION ( 'NONE',  ( 0.000000000000000000, 0.000000000000000000, -1.000000000000000000 ) ) ;
#3259=DIRECTION ( 'NONE',  ( -0.000000000000000000, -0.000000000000000000, 1.000000000000000000 ) ) ;
#3275=SHAPE_REPRESENTATION ( 'Vertical Telescoping Support Column', ( #4154 ), #5370 ) ;
#3279=PRODUCT_DEFINITION_FORMATION_WITH_SPECIFIED_SOURCE ( 'ANY', '', #1749, .NOT_KNOWN. ) ;
#3285=DIRECTION ( 'NONE',  ( 1.000000000000000000, 0.000000000000000000, 0.000000000000000000 ) ) ;
#3286=EDGE_CURVE ( 'NONE', #4279, #2752, #2321, .T. ) ;
#3290=ORIENTED_EDGE ( 'NONE', *, *, #1044, .F. ) ;
#3291=FACE_OUTER_BOUND ( 'NONE', #4091, .T. ) ;
#3308=CARTESIAN_POINT ( 'NONE',  ( 0.000000000000000000, 390.0000000000000000, 25.00000000000000000 ) ) ;
#3320=ORIENTED_EDGE ( 'NONE', *, *, #1212, .F. ) ;
#3334=FILL_AREA_STYLE_COLOUR ( '', #2501 ) ;
#3335=ORIENTED_EDGE ( 'NONE', *, *, #3667, .T. ) ;
#3336=ORIENTED_EDGE ( 'NONE', *, *, #2969, .F. ) ;
#3346=ADVANCED_FACE ( 'NONE', ( #1546 ), #4440, .F. ) ;
#3347=EDGE_LOOP ( 'NONE', ( #1302, #759, #5368, #1824 ) ) ;
#3350=CYLINDRICAL_SURFACE ( 'NONE', #3555, 6.499999999999988454 ) ;
#3425=EDGE_CURVE ( 'NONE', #871, #4239, #3728, .T. ) ;
#3433=DIRECTION ( 'NONE',  ( 0.000000000000000000, 0.000000000000000000, -1.000000000000000000 ) ) ;
#3435=ORIENTED_EDGE ( 'NONE', *, *, #4808, .T. ) ;
#3448=CARTESIAN_POINT ( 'NONE',  ( 0.000000000000000000, 510.0000000000000000, -25.00000000000000000 ) ) ;
#3464=VECTOR ( 'NONE', #4290, 999.9999999999998863 ) ;
#3473=FACE_OUTER_BOUND ( 'NONE', #398, .T. ) ;
#3478=CYLINDRICAL_SURFACE ( 'NONE', #5117, 6.499999999999988454 ) ;
#3480=EDGE_CURVE ( 'NONE', #1452, #2957, #1068, .T. ) ;
#3485=DIRECTION ( 'NONE',  ( 1.000000000000000000, 0.000000000000000000, 0.000000000000000000 ) ) ;
#3486=CARTESIAN_POINT ( 'NONE',  ( -6.499999999999988454, 450.0000000000000000, 25.00000000000000000 ) ) ;
#3489=VERTEX_POINT ( 'NONE', #956 ) ;
#3492=DIRECTION ( 'NONE',  ( -0.000000000000000000, -0.000000000000000000, 1.000000000000000000 ) ) ;
#3495=LINE ( 'NONE', #2647, #901 ) ;
#3499=DIRECTION ( 'NONE',  ( 0.000000000000000000, -0.000000000000000000, 1.000000000000000000 ) ) ;
#3508=CARTESIAN_POINT ( 'NONE',  ( -24.99999999999999645, 810.0000000000000000, -25.00000000000000000 ) ) ;
#3512=DIRECTION ( 'NONE',  ( -0.000000000000000000, -0.000000000000000000, 1.000000000000000000 ) ) ;
#3517=VERTEX_POINT ( 'NONE', #3042 ) ;
#3523=VECTOR ( 'NONE', #640, 1000.000000000000000 ) ;
#3527=CYLINDRICAL_SURFACE ( 'NONE', #5053, 6.499999999999988454 ) ;
#3531=FACE_OUTER_BOUND ( 'NONE', #610, .T. ) ;
#3532=AXIS2_PLACEMENT_3D ( 'NONE', #4955, #1563, #2064 ) ;
#3544=ORIENTED_EDGE ( 'NONE', *, *, #4879, .F. ) ;
#3545=LINE ( 'NONE', #2703, #472 ) ;
#3547=LINE ( 'NONE', #1394, #1211 ) ;
#3555=AXIS2_PLACEMENT_3D ( 'NONE', #2952, #2193, #4245 ) ;
#3562=DIRECTION ( 'NONE',  ( 1.000000000000000000, 0.000000000000000000, 0.000000000000000000 ) ) ;
#3566=PRODUCT_DEFINITION ( 'UNKNOWN', '', #3279, #5276 ) ;
#3567=DIRECTION ( 'NONE',  ( 1.000000000000000000, 0.000000000000000000, 0.000000000000000000 ) ) ;
#3569=VERTEX_POINT ( 'NONE', #1216 ) ;
#3572=VERTEX_POINT ( 'NONE', #1932 ) ;
#3582=CARTESIAN_POINT ( 'NONE',  ( 0.000000000000000000, 510.0000000000000000, 25.00000000000000000 ) ) ;
#3587=EDGE_LOOP ( 'NONE', ( #3902, #991 ) ) ;
#3598=EDGE_LOOP ( 'NONE', ( #765, #3247, #4474, #3335 ) ) ;
#3616=DIRECTION ( 'NONE',  ( 0.000000000000000000, -0.000000000000000000, 1.000000000000000000 ) ) ;
#3620=FACE_OUTER_BOUND ( 'NONE', #4070, .T. ) ;
#3652=DIRECTION ( 'NONE',  ( -0.000000000000000000, -0.000000000000000000, 1.000000000000000000 ) ) ;
#3659=ORIENTED_EDGE ( 'NONE', *, *, #5060, .F. ) ;
#3665=DIRECTION ( 'NONE',  ( 1.000000000000000000, 0.000000000000000000, 0.000000000000000000 ) ) ;
#3667=EDGE_CURVE ( 'NONE', #2863, #1641, #1355, .T. ) ;
#3671=DIRECTION ( 'NONE',  ( 1.000000000000000000, 0.000000000000000000, 0.000000000000000000 ) ) ;
#3679=DIRECTION ( 'NONE',  ( 0.000000000000000000, -0.000000000000000000, 1.000000000000000000 ) ) ;
#3691=ORIENTED_EDGE ( 'NONE', *, *, #3838, .T. ) ;
#3697=DIRECTION ( 'NONE',  ( 0.000000000000000000, -0.000000000000000000, 1.000000000000000000 ) ) ;
#3707=VECTOR ( 'NONE', #3080, 1000.000000000000000 ) ;
#3713=EDGE_LOOP ( 'NONE', ( #558, #816 ) ) ;
#3716=EDGE_LOOP ( 'NONE', ( #4373, #3110, #782, #2901 ) ) ;
#3723=ADVANCED_FACE ( 'NONE', ( #3853, #2261, #2648, #1766, #1870, #4697 ), #3113, .F. ) ;
#3724=ORIENTED_EDGE ( 'NONE', *, *, #5316, .T. ) ;
#3728=LINE ( 'NONE', #4735, #3464 ) ;
#3735=CARTESIAN_POINT ( 'NONE',  ( 0.000000000000000000, 390.0000000000000000, 25.00000000000000000 ) ) ;
#3745=CIRCLE ( 'NONE', #1446, 5.035999999999999588 ) ;
#3761=FACE_OUTER_BOUND ( 'NONE', #1200, .T. ) ;
#3768=CARTESIAN_POINT ( 'NONE',  ( 25.00000000000000000, 810.0000000000000000, 25.00000000000000711 ) ) ;
#3770=SURFACE_STYLE_USAGE ( .BOTH. , #4123 ) ;
#3782=ADVANCED_FACE ( 'NONE', ( #2604 ), #3957, .T. ) ;
#3784=ORIENTED_EDGE ( 'NONE', *, *, #3425, .T. ) ;
#3785=DIRECTION ( 'NONE',  ( 0.000000000000000000, 0.000000000000000000, 1.000000000000000000 ) ) ;
#3811=CARTESIAN_POINT ( 'NONE',  ( 25.00000000000000000, 810.0000000000000000, 25.00000000000000711 ) ) ;
#3819=( LENGTH_UNIT ( ) NAMED_UNIT ( * ) SI_UNIT ( .MILLI., .METRE. ) );
#3823=FACE_BOUND ( 'NONE', #3713, .T. ) ;
#3838=EDGE_CURVE ( 'NONE', #791, #4561, #1201, .T. ) ;
#3847=DIRECTION ( 'NONE',  ( 1.000000000000000000, 0.000000000000000000, 0.000000000000000000 ) ) ;
#3853=FACE_BOUND ( 'NONE', #3587, .T. ) ;
#3855=ADVANCED_FACE ( 'NONE', ( #3159 ), #774, .T. ) ;
#3868=ORIENTED_EDGE ( 'NONE', *, *, #1980, .F. ) ;
#3887=CARTESIAN_POINT ( 'NONE',  ( 0.000000000000000000, 570.0000000000000000, 25.00000000000000000 ) ) ;
#3889=AXIS2_PLACEMENT_3D ( 'NONE', #985, #1807, #2297 ) ;
#3902=ORIENTED_EDGE ( 'NONE', *, *, #5027, .T. ) ;
#3905=CIRCLE ( 'NONE', #1291, 5.999999999999996447 ) ;
#3922=ORIENTED_EDGE ( 'NONE', *, *, #4856, .F. ) ;
#3926=CARTESIAN_POINT ( 'NONE',  ( -6.499999999999988454, 510.0000000000000000, -25.00000000000000000 ) ) ;
#3938=DIRECTION ( 'NONE',  ( 0.000000000000000000, 0.000000000000000000, 1.000000000000000000 ) ) ;
#3944=EDGE_CURVE ( 'NONE', #2006, #3569, #2521, .T. ) ;
#3947=ORIENTED_EDGE ( 'NONE', *, *, #2279, .F. ) ;
#3949=ORIENTED_EDGE ( 'NONE', *, *, #1592, .F. ) ;
#3951=ORIENTED_EDGE ( 'NONE', *, *, #4487, .T. ) ;
#3957=PLANE ( 'NONE',  #4167 ) ;
#3964=CARTESIAN_POINT ( 'NONE',  ( 0.000000000000000000, 810.0000000000000000, 0.000000000000000000 ) ) ;
#3972=EDGE_CURVE ( 'NONE', #838, #1279, #2883, .T. ) ;
#3982=VECTOR ( 'NONE', #164, 1000.000000000000000 ) ;
#3993=AXIS2_PLACEMENT_3D ( 'NONE', #2052, #3679, #749 ) ;
#3998=CIRCLE ( 'NONE', #4945, 6.499999999999988454 ) ;
#4007=CONICAL_SURFACE ( 'NONE', #2339, 5.999999999999996447, 0.7853981633974074228 ) ;
#4010=ORIENTED_EDGE ( 'NONE', *, *, #4084, .T. ) ;
#4013=ORIENTED_EDGE ( 'NONE', *, *, #3944, .T. ) ;
#4014=CARTESIAN_POINT ( 'NONE',  ( 0.000000000000000000, 839.0360000000000582, -5.999999999999996447 ) ) ;
#4017=CARTESIAN_POINT ( 'NONE',  ( -6.499999999999988454, 390.0000000000000000, -25.00000000000000000 ) ) ;
#4054=CARTESIAN_POINT ( 'NONE',  ( -6.499999999999988454, 390.0000000000000000, 25.00000000000000000 ) ) ;
#4063=CARTESIAN_POINT ( 'NONE',  ( 7.347880794884115792E-16, 839.0360000000000582, 5.999999999999996447 ) ) ;
#4070=EDGE_LOOP ( 'NONE', ( #3320, #1751, #2933, #3691 ) ) ;
#4075=VECTOR ( 'NONE', #1129, 1000.000000000000000 ) ;
#4077=VERTEX_POINT ( 'NONE', #1051 ) ;
#4082=SHAPE_DEFINITION_REPRESENTATION ( #493, #3275 ) ;
#4084=EDGE_CURVE ( 'NONE', #4077, #1160, #4644, .T. ) ;
#4085=DIRECTION ( 'NONE',  ( 1.000000000000000000, 0.000000000000000000, 0.000000000000000000 ) ) ;
#4091=EDGE_LOOP ( 'NONE', ( #693, #3784, #3868, #396 ) ) ;
#4106=DIRECTION ( 'NONE',  ( -0.000000000000000000, -0.000000000000000000, 1.000000000000000000 ) ) ;
#4107=CARTESIAN_POINT ( 'NONE',  ( 0.000000000000000000, 570.0000000000000000, -25.00000000000000000 ) ) ;
#4113=CARTESIAN_POINT ( 'NONE',  ( 0.000000000000000000, 390.0000000000000000, 25.00000000000000000 ) ) ;
#4123=SURFACE_SIDE_STYLE ('',( #2141 ) ) ;
#4154=AXIS2_PLACEMENT_3D ( 'NONE', #2434, #5290, #769 ) ;
#4167=AXIS2_PLACEMENT_3D ( 'NONE', #210, #5100, #3081 ) ;
#4173=ORIENTED_EDGE ( 'NONE', *, *, #4627, .F. ) ;
#4175=ORIENTED_EDGE ( 'NONE', *, *, #2969, .T. ) ;
#4184=DIRECTION ( 'NONE',  ( 0.000000000000000000, 0.000000000000000000, -1.000000000000000000 ) ) ;
#4187=ORIENTED_EDGE ( 'NONE', *, *, #4084, .F. ) ;
#4199=DIRECTION ( 'NONE',  ( -0.000000000000000000, -0.000000000000000000, 1.000000000000000000 ) ) ;
#4221=MECHANICAL_DESIGN_GEOMETRIC_PRESENTATION_REPRESENTATION('',(#4912),#1855);
#4224=DIRECTION ( 'NONE',  ( -0.000000000000000000, -1.000000000000000000, -0.000000000000000000 ) ) ;
#4227=CIRCLE ( 'NONE', #1858, 6.000000000000000000 ) ;
#4232=DIRECTION ( 'NONE',  ( -0.000000000000000000, -0.000000000000000000, 1.000000000000000000 ) ) ;
#4239=VERTEX_POINT ( 'NONE', #4063 ) ;
#4245=DIRECTION ( 'NONE',  ( 1.000000000000000000, 0.000000000000000000, 0.000000000000000000 ) ) ;
#4248=AXIS2_PLACEMENT_3D ( 'NONE', #355, #2440, #269 ) ;
#4254=CARTESIAN_POINT ( 'NONE',  ( 0.000000000000000000, 810.0000000000000000, -5.999999999999998224 ) ) ;
#4257=CYLINDRICAL_SURFACE ( 'NONE', #780, 6.499999999999988454 ) ;
#4262=CYLINDRICAL_SURFACE ( 'NONE', #2762, 6.499999999999988454 ) ;
#4275=CARTESIAN_POINT ( 'NONE',  ( 0.000000000000000000, 510.0000000000000000, 25.00000000000000000 ) ) ;
#4279=VERTEX_POINT ( 'NONE', #5312 ) ;
#4290=DIRECTION ( 'NONE',  ( 8.659560562354580336E-17, -0.7071067811865765496, 0.7071067811865185959 ) ) ;
#4304=EDGE_LOOP ( 'NONE', ( #2424, #4352 ) ) ;
#4305=VECTOR ( 'NONE', #746, 1000.000000000000000 ) ;
#4308=CARTESIAN_POINT ( 'NONE',  ( 25.00000000000000000, 810.0000000000000000, -25.00000000000000000 ) ) ;
#4314=ADVANCED_FACE ( 'NONE', ( #4915 ), #725, .F. ) ;
#4320=DIRECTION ( 'NONE',  ( -0.000000000000000000, -0.000000000000000000, 1.000000000000000000 ) ) ;
#4328=VECTOR ( 'NONE', #4399, 1000.000000000000000 ) ;
#4334=ORIENTED_EDGE ( 'NONE', *, *, #2160, .T. ) ;
#4335=VERTEX_POINT ( 'NONE', #1368 ) ;
#4342=DIRECTION ( 'NONE',  ( 0.000000000000000000, 0.000000000000000000, -1.000000000000000000 ) ) ;
#4352=ORIENTED_EDGE ( 'NONE', *, *, #3286, .T. ) ;
#4356=CARTESIAN_POINT ( 'NONE',  ( -6.499999999999988454, 510.0000000000000000, 25.00000000000000000 ) ) ;
#4362=ADVANCED_FACE ( 'NONE', ( #1776 ), #3350, .F. ) ;
#4373=ORIENTED_EDGE ( 'NONE', *, *, #2876, .F. ) ;
#4386=DIRECTION ( 'NONE',  ( 0.000000000000000000, -0.000000000000000000, 1.000000000000000000 ) ) ;
#4394=DIRECTION ( 'NONE',  ( 0.000000000000000000, 0.000000000000000000, -1.000000000000000000 ) ) ;
#4396=AXIS2_PLACEMENT_3D ( 'NONE', #1246, #4456, #3665 ) ;
#4399=DIRECTION ( 'NONE',  ( -6.938893903907228378E-17, 0.000000000000000000, 1.000000000000000000 ) ) ;
#4419=DIRECTION ( 'NONE',  ( 0.000000000000000000, 1.000000000000000000, -0.000000000000000000 ) ) ;
#4428=VERTEX_POINT ( 'NONE', #1850 ) ;
#4440=CYLINDRICAL_SURFACE ( 'NONE', #4840, 6.499999999999988454 ) ;
#4441=DIRECTION ( 'NONE',  ( -0.000000000000000000, -1.000000000000000000, -0.000000000000000000 ) ) ;
#4456=DIRECTION ( 'NONE',  ( -0.000000000000000000, -0.000000000000000000, 1.000000000000000000 ) ) ;
#4461=CARTESIAN_POINT ( 'NONE',  ( 6.499999999999988454, 510.0000000000000000, -25.00000000000000000 ) ) ;
#4474=ORIENTED_EDGE ( 'NONE', *, *, #4566, .T. ) ;
#4482=ORIENTED_EDGE ( 'NONE', *, *, #4540, .T. ) ;
#4487=EDGE_CURVE ( 'NONE', #5257, #5200, #2659, .T. ) ;
#4492=ORIENTED_EDGE ( 'NONE', *, *, #2792, .T. ) ;
#4499=ADVANCED_FACE ( 'NONE', ( #3531 ), #1885, .T. ) ;
#4508=AXIS2_PLACEMENT_3D ( 'NONE', #3448, #3499, #975 ) ;
#4526=FACE_OUTER_BOUND ( 'NONE', #2729, .T. ) ;
#4527=CARTESIAN_POINT ( 'NONE',  ( -25.00000000000000000, 210.0000000000000284, 24.99999999999999645 ) ) ;
#4528=CARTESIAN_POINT ( 'NONE',  ( 25.00000000000000000, 810.0000000000000000, 25.00000000000000711 ) ) ;
#4537=DIRECTION ( 'NONE',  ( -0.000000000000000000, -0.000000000000000000, 1.000000000000000000 ) ) ;
#4540=EDGE_CURVE ( 'NONE', #2438, #3240, #1536, .T. ) ;
#4541=ORIENTED_EDGE ( 'NONE', *, *, #3667, .F. ) ;
#4553=VERTEX_POINT ( 'NONE', #2246 ) ;
#4561=VERTEX_POINT ( 'NONE', #3486 ) ;
#4566=EDGE_CURVE ( 'NONE', #3517, #2863, #4708, .T. ) ;
#4572=CARTESIAN_POINT ( 'NONE',  ( 6.499999999999988454, 450.0000000000000000, 25.00000000000000000 ) ) ;
#4573=CARTESIAN_POINT ( 'NONE',  ( 6.499999999999988454, 510.0000000000000000, 25.00000000000000000 ) ) ;
#4590=ORIENTED_EDGE ( 'NONE', *, *, #2621, .T. ) ;
#4597=EDGE_CURVE ( 'NONE', #3517, #752, #931, .T. ) ;
#4611=PLANE ( 'NONE',  #1781 ) ;
#4613=ORIENTED_EDGE ( 'NONE', *, *, #2776, .F. ) ;
#4618=CARTESIAN_POINT ( 'NONE',  ( -25.00000000000000000, 810.0000000000000000, 24.99999999999999645 ) ) ;
#4626=LINE ( 'NONE', #5076, #1610 ) ;
#4627=EDGE_CURVE ( 'NONE', #2006, #1452, #2895, .T. ) ;
#4644=LINE ( 'NONE', #3508, #4328 ) ;
#4681=EDGE_LOOP ( 'NONE', ( #3724, #5148 ) ) ;
#4686=DIRECTION ( 'NONE',  ( -0.000000000000000000, -0.000000000000000000, 1.000000000000000000 ) ) ;
#4697=FACE_BOUND ( 'NONE', #1648, .T. ) ;
#4702=ORIENTED_EDGE ( 'NONE', *, *, #3425, .F. ) ;
#4705=DIRECTION ( 'NONE',  ( -0.000000000000000000, -0.000000000000000000, 1.000000000000000000 ) ) ;
#4708=LINE ( 'NONE', #5137, #2959 ) ;
#4709=DIRECTION ( 'NONE',  ( -0.000000000000000000, -0.000000000000000000, 1.000000000000000000 ) ) ;
#4710=( NAMED_UNIT ( * ) SI_UNIT ( $, .STERADIAN. ) SOLID_ANGLE_UNIT ( ) );
#4721=EDGE_LOOP ( 'NONE', ( #2871, #1330 ) ) ;
#4735=CARTESIAN_POINT ( 'NONE',  ( 7.347880794884115792E-16, 839.0360000000000582, 5.999999999999996447 ) ) ;
#4741=VECTOR ( 'NONE', #2215, 1000.000000000000000 ) ;
#4744=SHAPE_REPRESENTATION_RELATIONSHIP ( 'NONE' , 'NONE' ,  #3275, #119 ) ;
#4750=DIRECTION ( 'NONE',  ( -0.000000000000000000, -0.000000000000000000, 1.000000000000000000 ) ) ;
#4767=CARTESIAN_POINT ( 'NONE',  ( -6.499999999999988454, 330.0000000000000000, -25.00000000000000000 ) ) ;
#4794=EDGE_LOOP ( 'NONE', ( #1999, #3336, #4187, #4917 ) ) ;
#4808=EDGE_CURVE ( 'NONE', #871, #3246, #3745, .T. ) ;
#4809=ORIENTED_EDGE ( 'NONE', *, *, #1736, .F. ) ;
#4838=ORIENTED_EDGE ( 'NONE', *, *, #2265, .F. ) ;
#4840=AXIS2_PLACEMENT_3D ( 'NONE', #1988, #5297, #3671 ) ;
#4850=CIRCLE ( 'NONE', #423, 6.499999999999988454 ) ;
#4856=EDGE_CURVE ( 'NONE', #5257, #838, #1369, .T. ) ;
#4857=EDGE_CURVE ( 'NONE', #2752, #3572, #186, .T. ) ;
#4877=PRODUCT_CONTEXT ( 'NONE', #5230, 'mechanical' ) ;
#4879=EDGE_CURVE ( 'NONE', #4553, #2728, #1542, .T. ) ;
#4889=DIRECTION ( 'NONE',  ( -0.000000000000000000, -0.000000000000000000, 1.000000000000000000 ) ) ;
#4896=ADVANCED_FACE ( 'NONE', ( #1799 ), #3478, .F. ) ;
#4905=CARTESIAN_POINT ( 'NONE',  ( 25.00000000000000000, 210.0000000000000284, -25.00000000000000000 ) ) ;
#4908=LINE ( 'NONE', #2020, #5064 ) ;
#4912=STYLED_ITEM('',(#5412),#1812);
#4915=FACE_OUTER_BOUND ( 'NONE', #869, .T. ) ;
#4917=ORIENTED_EDGE ( 'NONE', *, *, #5224, .T. ) ;
#4933=DIRECTION ( 'NONE',  ( 1.000000000000000000, 0.000000000000000000, 0.000000000000000000 ) ) ;
#4945=AXIS2_PLACEMENT_3D ( 'NONE', #3582, #2376, #357 ) ;
#4949=CIRCLE ( 'NONE', #1448, 6.499999999999988454 ) ;
#4950=ORIENTED_EDGE ( 'NONE', *, *, #4808, .F. ) ;
#4955=CARTESIAN_POINT ( 'NONE',  ( 0.000000000000000000, 839.0360000000000582, 0.000000000000000000 ) ) ;
#4964=( NAMED_UNIT ( * ) PLANE_ANGLE_UNIT ( ) SI_UNIT ( $, .RADIAN. ) );
#4981=EDGE_CURVE ( 'NONE', #5200, #1279, #3998, .T. ) ;
#4982=VERTEX_POINT ( 'NONE', #271 ) ;
#4984=PRESENTATION_STYLE_ASSIGNMENT (( #3770 ) ) ;
#4996=AXIS2_PLACEMENT_3D ( 'NONE', #4618, #84, #944 ) ;
#5000=ORIENTED_EDGE ( 'NONE', *, *, #2621, .F. ) ;
#5016=AXIS2_PLACEMENT_3D ( 'NONE', #1849, #1409, #253 ) ;
#5027=EDGE_CURVE ( 'NONE', #838, #5257, #4850, .T. ) ;
#5041=DIRECTION ( 'NONE',  ( -0.000000000000000000, -1.000000000000000000, -0.000000000000000000 ) ) ;
#5053=AXIS2_PLACEMENT_3D ( 'NONE', #2383, #3652, #1097 ) ;
#5060=EDGE_CURVE ( 'NONE', #4239, #2365, #3905, .T. ) ;
#5064=VECTOR ( 'NONE', #2821, 1000.000000000000000 ) ;
#5067=DIRECTION ( 'NONE',  ( 0.000000000000000000, 0.000000000000000000, -1.000000000000000000 ) ) ;
#5075=DIRECTION ( 'NONE',  ( -0.000000000000000000, -0.000000000000000000, 1.000000000000000000 ) ) ;
#5076=CARTESIAN_POINT ( 'NONE',  ( -25.00000000000000000, 810.0000000000000000, 24.99999999999999645 ) ) ;
#5090=FACE_BOUND ( 'NONE', #5345, .T. ) ;
#5093=CLOSED_SHELL ( 'NONE', ( #4362, #2581, #408, #452, #223, #4896, #3346, #2051, #1926, #2391, #1331, #930, #2493, #3723, #237, #4314, #3782, #4499, #3855, #543, #5206 ) ) ;
#5099=DIRECTION ( 'NONE',  ( 0.000000000000000000, -0.000000000000000000, 1.000000000000000000 ) ) ;
#5100=DIRECTION ( 'NONE',  ( 0.000000000000000000, 1.000000000000000000, 0.000000000000000000 ) ) ;
#5101=DIRECTION ( 'NONE',  ( -0.000000000000000000, -1.000000000000000000, -0.000000000000000000 ) ) ;
#5103=CARTESIAN_POINT ( 'NONE',  ( 6.499999999999988454, 570.0000000000000000, 25.00000000000000000 ) ) ;
#5112=VECTOR ( 'NONE', #4199, 1000.000000000000000 ) ;
#5117=AXIS2_PLACEMENT_3D ( 'NONE', #3061, #3037, #2733 ) ;
#5121=PLANE ( 'NONE',  #4996 ) ;
#5122=FACE_OUTER_BOUND ( 'NONE', #2973, .T. ) ;
#5137=CARTESIAN_POINT ( 'NONE',  ( 6.499999999999988454, 390.0000000000000000, 25.00000000000000000 ) ) ;
#5148=ORIENTED_EDGE ( 'NONE', *, *, #2876, .T. ) ;
#5171=DIRECTION ( 'NONE',  ( 0.000000000000000000, -0.000000000000000000, 1.000000000000000000 ) ) ;
#5179=DIRECTION ( 'NONE',  ( -0.000000000000000000, -1.000000000000000000, -0.000000000000000000 ) ) ;
#5198=EDGE_CURVE ( 'NONE', #1279, #5200, #1639, .T. ) ;
#5200=VERTEX_POINT ( 'NONE', #4356 ) ;
#5206=ADVANCED_FACE ( 'NONE', ( #5122 ), #4257, .F. ) ;
#5208=CARTESIAN_POINT ( 'NONE',  ( 25.00000000000000000, 210.0000000000000284, 25.00000000000000711 ) ) ;
#5212=DIRECTION ( 'NONE',  ( -0.000000000000000000, -0.000000000000000000, 1.000000000000000000 ) ) ;
#5220=DIRECTION ( 'NONE',  ( -0.000000000000000000, -1.000000000000000000, -0.000000000000000000 ) ) ;
#5224=EDGE_CURVE ( 'NONE', #4077, #3489, #3547, .T. ) ;
#5228=LINE ( 'NONE', #3075, #3523 ) ;
#5230=APPLICATION_CONTEXT ( 'automotive_design' ) ;
#5242=EDGE_CURVE ( 'NONE', #4561, #791, #4949, .T. ) ;
#5249=CARTESIAN_POINT ( 'NONE',  ( 6.499999999999988454, 570.0000000000000000, -25.00000000000000000 ) ) ;
#5257=VERTEX_POINT ( 'NONE', #3926 ) ;
#5265=CIRCLE ( 'NONE', #3172, 5.035999999999999588 ) ;
#5276=PRODUCT_DEFINITION_CONTEXT ( 'detailed design', #19, 'design' ) ;
#5290=DIRECTION ( 'NONE',  ( 0.000000000000000000, 0.000000000000000000, 1.000000000000000000 ) ) ;
#5296=DIRECTION ( 'NONE',  ( 1.000000000000000000, 0.000000000000000000, 0.000000000000000000 ) ) ;
#5297=DIRECTION ( 'NONE',  ( -0.000000000000000000, -0.000000000000000000, 1.000000000000000000 ) ) ;
#5304=DIRECTION ( 'NONE',  ( -1.000000000000000000, 0.000000000000000000, 0.000000000000000000 ) ) ;
#5312=CARTESIAN_POINT ( 'NONE',  ( -6.499999999999988454, 570.0000000000000000, -25.00000000000000000 ) ) ;
#5316=EDGE_CURVE ( 'NONE', #4982, #4428, #2161, .T. ) ;
#5318=FACE_OUTER_BOUND ( 'NONE', #3598, .T. ) ;
#5345=EDGE_LOOP ( 'NONE', ( #4838, #1652 ) ) ;
#5349=CARTESIAN_POINT ( 'NONE',  ( 0.000000000000000000, 840.0000000000001137, -5.035999999999999588 ) ) ;
#5368=ORIENTED_EDGE ( 'NONE', *, *, #194, .T. ) ;
#5370=( GEOMETRIC_REPRESENTATION_CONTEXT ( 3 ) GLOBAL_UNCERTAINTY_ASSIGNED_CONTEXT ( ( #95 ) ) GLOBAL_UNIT_ASSIGNED_CONTEXT ( ( #3819, #2879, #456 ) ) REPRESENTATION_CONTEXT ( 'NONE', 'WORKASPACE' ) );
#5386=ORIENTED_EDGE ( 'NONE', *, *, #3944, .F. ) ;
#5406=COLOUR_RGB('Light Blue',0.38,0.62,0.78);
#5407=FILL_AREA_STYLE_COLOUR('',#5406);
#5408=FILL_AREA_STYLE('',(#5407));
#5409=SURFACE_STYLE_FILL_AREA(#5408);
#5410=SURFACE_SIDE_STYLE('',(#5409));
#5411=SURFACE_STYLE_USAGE(.BOTH.,#5410);
#5412=PRESENTATION_STYLE_ASSIGNMENT((#5411));
ENDSEC;
END-ISO-10303-21;
